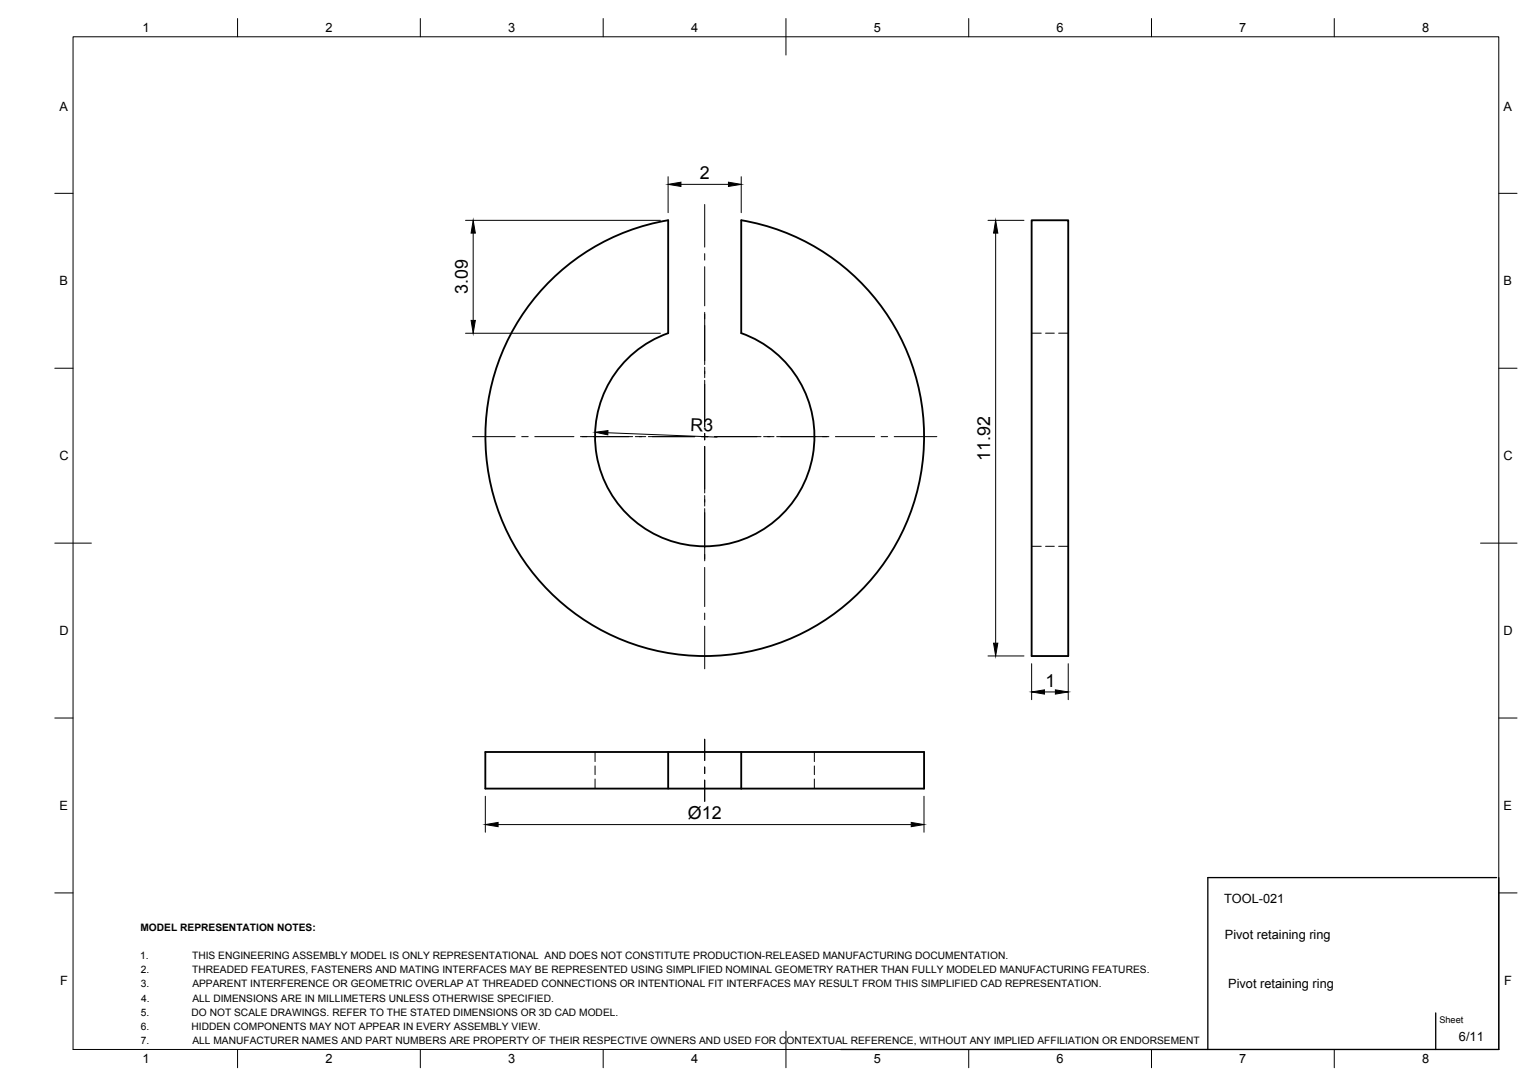
ISO-10303-21;
HEADER;
/* Generated by software containing ST-Developer
 * from STEP Tools, Inc. (www.steptools.com) 
 */

FILE_DESCRIPTION(
/* description */ (''),
/* implementation_level */ '2;1');

FILE_NAME(
/* name */ 'Pivot retaining ring.step',
/* time_stamp */ '2026-11-10T09:05:57-08:00',
/* author */ (''),
/* organization */ (''),
/* preprocessor_version */ 'ST-DEVELOPER v20.2',
/* originating_system */ 'Autodesk Translation Framework v15.17.0.0',
/* authorisation */ '');

FILE_SCHEMA (('AUTOMOTIVE_DESIGN { 1 0 10303 214 3 1 1 }'));
ENDSEC;

DATA;
#10=MECHANICAL_DESIGN_GEOMETRIC_PRESENTATION_REPRESENTATION('',(#568),#19618);
#548=SHAPE_REPRESENTATION_RELATIONSHIP('SRR','None',#19667,#558);
#558=ADVANCED_BREP_SHAPE_REPRESENTATION('',(#578),#19610);
#568=STYLED_ITEM('',(#19730),#578);
#578=MANIFOLD_SOLID_BREP('Body1',#7106);
#703=PLANE('',#7362);
#704=PLANE('',#7363);
#705=PLANE('',#7364);
#706=PLANE('',#7371);
#892=FACE_OUTER_BOUND('',#1314,.T.);
#893=FACE_OUTER_BOUND('',#1315,.T.);
#894=FACE_OUTER_BOUND('',#1316,.T.);
#895=FACE_OUTER_BOUND('',#1317,.T.);
#896=FACE_OUTER_BOUND('',#1318,.T.);
#897=FACE_OUTER_BOUND('',#1319,.T.);
#1314=EDGE_LOOP('',(#4866,#4867,#4868,#4869));
#1315=EDGE_LOOP('',(#4870,#4871,#4872,#4873));
#1316=EDGE_LOOP('',(#4874,#4875,#4876,#4877));
#1317=EDGE_LOOP('',(#4878,#4879,#4880,#4881));
#1318=EDGE_LOOP('',(#4882,#4883,#4884,#4885));
#1319=EDGE_LOOP('',(#4886,#4887,#4888,#4889));
#1817=LINE('',#9697,#2276);
#1818=LINE('',#9699,#2277);
#1819=LINE('',#9701,#2278);
#1820=LINE('',#9702,#2279);
#1821=LINE('',#9706,#2280);
#1822=LINE('',#9708,#2281);
#1823=LINE('',#9710,#2282);
#1824=LINE('',#9711,#2283);
#2276=VECTOR('',#8166,1.);
#2277=VECTOR('',#8167,1.);
#2278=VECTOR('',#8168,1.);
#2279=VECTOR('',#8169,1.);
#2280=VECTOR('',#8172,1.);
#2281=VECTOR('',#8173,1.);
#2282=VECTOR('',#8174,1.);
#2283=VECTOR('',#8175,1.);
#2678=CIRCLE('',#7365,0.6);
#2679=CIRCLE('',#7366,0.3);
#2680=CIRCLE('',#7368,0.3);
#2681=CIRCLE('',#7370,0.6);
#2929=VERTEX_POINT('',#9695);
#2930=VERTEX_POINT('',#9696);
#2931=VERTEX_POINT('',#9698);
#2932=VERTEX_POINT('',#9700);
#2933=VERTEX_POINT('',#9704);
#2934=VERTEX_POINT('',#9705);
#2935=VERTEX_POINT('',#9707);
#2936=VERTEX_POINT('',#9709);
#3658=EDGE_CURVE('',#2929,#2930,#1817,.T.);
#3659=EDGE_CURVE('',#2931,#2929,#1818,.T.);
#3660=EDGE_CURVE('',#2932,#2931,#1819,.T.);
#3661=EDGE_CURVE('',#2930,#2932,#1820,.T.);
#3662=EDGE_CURVE('',#2933,#2934,#1821,.T.);
#3663=EDGE_CURVE('',#2935,#2933,#1822,.T.);
#3664=EDGE_CURVE('',#2936,#2935,#1823,.T.);
#3665=EDGE_CURVE('',#2934,#2936,#1824,.T.);
#3666=EDGE_CURVE('',#2931,#2936,#2678,.T.);
#3667=EDGE_CURVE('',#2934,#2929,#2679,.T.);
#3668=EDGE_CURVE('',#2933,#2930,#2680,.T.);
#3669=EDGE_CURVE('',#2932,#2935,#2681,.T.);
#4866=ORIENTED_EDGE('',*,*,#3658,.F.);
#4867=ORIENTED_EDGE('',*,*,#3659,.F.);
#4868=ORIENTED_EDGE('',*,*,#3660,.F.);
#4869=ORIENTED_EDGE('',*,*,#3661,.F.);
#4870=ORIENTED_EDGE('',*,*,#3662,.F.);
#4871=ORIENTED_EDGE('',*,*,#3663,.F.);
#4872=ORIENTED_EDGE('',*,*,#3664,.F.);
#4873=ORIENTED_EDGE('',*,*,#3665,.F.);
#4874=ORIENTED_EDGE('',*,*,#3665,.T.);
#4875=ORIENTED_EDGE('',*,*,#3666,.F.);
#4876=ORIENTED_EDGE('',*,*,#3659,.T.);
#4877=ORIENTED_EDGE('',*,*,#3667,.F.);
#4878=ORIENTED_EDGE('',*,*,#3662,.T.);
#4879=ORIENTED_EDGE('',*,*,#3667,.T.);
#4880=ORIENTED_EDGE('',*,*,#3658,.T.);
#4881=ORIENTED_EDGE('',*,*,#3668,.F.);
#4882=ORIENTED_EDGE('',*,*,#3664,.T.);
#4883=ORIENTED_EDGE('',*,*,#3669,.F.);
#4884=ORIENTED_EDGE('',*,*,#3660,.T.);
#4885=ORIENTED_EDGE('',*,*,#3666,.T.);
#4886=ORIENTED_EDGE('',*,*,#3663,.T.);
#4887=ORIENTED_EDGE('',*,*,#3668,.T.);
#4888=ORIENTED_EDGE('',*,*,#3661,.T.);
#4889=ORIENTED_EDGE('',*,*,#3669,.T.);
#6583=CYLINDRICAL_SURFACE('',#7367,0.3);
#6584=CYLINDRICAL_SURFACE('',#7369,0.6);
#6771=ADVANCED_FACE('',(#892),#703,.F.);
#6772=ADVANCED_FACE('',(#893),#704,.F.);
#6773=ADVANCED_FACE('',(#894),#705,.F.);
#6774=ADVANCED_FACE('',(#895),#6583,.F.);
#6775=ADVANCED_FACE('',(#896),#6584,.T.);
#6776=ADVANCED_FACE('',(#897),#706,.T.);
#7106=CLOSED_SHELL('',(#6771,#6772,#6773,#6774,#6775,#6776));
#7361=AXIS2_PLACEMENT_3D('',#9693,#8162,#8163);
#7362=AXIS2_PLACEMENT_3D('',#9694,#8164,#8165);
#7363=AXIS2_PLACEMENT_3D('',#9703,#8170,#8171);
#7364=AXIS2_PLACEMENT_3D('',#9712,#8176,#8177);
#7365=AXIS2_PLACEMENT_3D('',#9713,#8178,#8179);
#7366=AXIS2_PLACEMENT_3D('',#9714,#8180,#8181);
#7367=AXIS2_PLACEMENT_3D('',#9715,#8182,#8183);
#7368=AXIS2_PLACEMENT_3D('',#9716,#8184,#8185);
#7369=AXIS2_PLACEMENT_3D('',#9717,#8186,#8187);
#7370=AXIS2_PLACEMENT_3D('',#9718,#8188,#8189);
#7371=AXIS2_PLACEMENT_3D('',#9719,#8190,#8191);
#8162=DIRECTION('axis',(0.,0.,1.));
#8163=DIRECTION('refdir',(1.,0.,0.));
#8164=DIRECTION('center_axis',(-1.,0.,0.));
#8165=DIRECTION('ref_axis',(0.,1.,0.));
#8166=DIRECTION('',(0.,0.,1.));
#8167=DIRECTION('',(0.,-1.,0.));
#8168=DIRECTION('',(0.,0.,-1.));
#8169=DIRECTION('',(0.,1.,0.));
#8170=DIRECTION('center_axis',(1.,0.,0.));
#8171=DIRECTION('ref_axis',(0.,-1.,0.));
#8172=DIRECTION('',(0.,0.,-1.));
#8173=DIRECTION('',(0.,-1.,0.));
#8174=DIRECTION('',(0.,0.,1.));
#8175=DIRECTION('',(0.,1.,0.));
#8176=DIRECTION('center_axis',(0.,0.,1.));
#8177=DIRECTION('ref_axis',(1.,0.,0.));
#8178=DIRECTION('center_axis',(0.,0.,1.));
#8179=DIRECTION('ref_axis',(1.,0.,0.));
#8180=DIRECTION('center_axis',(0.,0.,-1.));
#8181=DIRECTION('ref_axis',(1.,0.,0.));
#8182=DIRECTION('center_axis',(0.,0.,1.));
#8183=DIRECTION('ref_axis',(6.12323399573677E-17,-1.,0.));
#8184=DIRECTION('center_axis',(0.,0.,-1.));
#8185=DIRECTION('ref_axis',(1.,0.,0.));
#8186=DIRECTION('center_axis',(0.,0.,1.));
#8187=DIRECTION('ref_axis',(6.12323399573677E-17,-1.,0.));
#8188=DIRECTION('center_axis',(0.,0.,1.));
#8189=DIRECTION('ref_axis',(1.,0.,0.));
#8190=DIRECTION('center_axis',(0.,0.,1.));
#8191=DIRECTION('ref_axis',(1.,0.,0.));
#9693=CARTESIAN_POINT('',(0.,0.,0.));
#9694=CARTESIAN_POINT('Origin',(-0.1,0.,0.1));
#9695=CARTESIAN_POINT('',(-0.1,0.282842712474619,0.));
#9696=CARTESIAN_POINT('',(-0.1,0.282842712474619,0.1));
#9697=CARTESIAN_POINT('',(-0.1,0.282842712474619,0.));
#9698=CARTESIAN_POINT('',(-0.1,0.591607978309962,0.));
#9699=CARTESIAN_POINT('',(-0.1,0.,0.));
#9700=CARTESIAN_POINT('',(-0.1,0.591607978309962,0.1));
#9701=CARTESIAN_POINT('',(-0.1,0.591607978309962,0.));
#9702=CARTESIAN_POINT('',(-0.1,0.,0.1));
#9703=CARTESIAN_POINT('Origin',(0.1,1.2,0.1));
#9704=CARTESIAN_POINT('',(0.1,0.282842712474619,0.1));
#9705=CARTESIAN_POINT('',(0.1,0.282842712474619,0.));
#9706=CARTESIAN_POINT('',(0.1,0.282842712474619,0.));
#9707=CARTESIAN_POINT('',(0.1,0.591607978309962,0.1));
#9708=CARTESIAN_POINT('',(0.1,0.6,0.1));
#9709=CARTESIAN_POINT('',(0.1,0.591607978309962,0.));
#9710=CARTESIAN_POINT('',(0.1,0.591607978309962,0.));
#9711=CARTESIAN_POINT('',(0.1,0.6,0.));
#9712=CARTESIAN_POINT('Origin',(0.,0.,0.));
#9713=CARTESIAN_POINT('Origin',(0.,0.,0.));
#9714=CARTESIAN_POINT('Origin',(0.,0.,0.));
#9715=CARTESIAN_POINT('Origin',(0.,0.,0.));
#9716=CARTESIAN_POINT('Origin',(0.,0.,0.1));
#9717=CARTESIAN_POINT('Origin',(0.,0.,0.));
#9718=CARTESIAN_POINT('Origin',(0.,0.,0.1));
#9719=CARTESIAN_POINT('Origin',(0.,0.,0.1));
#19597=UNCERTAINTY_MEASURE_WITH_UNIT(LENGTH_MEASURE(0.001),#19619,
'DISTANCE_ACCURACY_VALUE',
'Maximum model space distance between geometric entities at asserted c
onnectivities');
#19605=UNCERTAINTY_MEASURE_WITH_UNIT(LENGTH_MEASURE(0.001),#19619,
'DISTANCE_ACCURACY_VALUE',
'Maximum model space distance between geometric entities at asserted c
onnectivities');
#19610=(
GEOMETRIC_REPRESENTATION_CONTEXT(3)
GLOBAL_UNCERTAINTY_ASSIGNED_CONTEXT((#19597))
GLOBAL_UNIT_ASSIGNED_CONTEXT((#19619,#19621,#19622))
REPRESENTATION_CONTEXT('','3D')
);
#19618=(
GEOMETRIC_REPRESENTATION_CONTEXT(3)
GLOBAL_UNCERTAINTY_ASSIGNED_CONTEXT((#19605))
GLOBAL_UNIT_ASSIGNED_CONTEXT((#19619,#19621,#19622))
REPRESENTATION_CONTEXT('','3D')
);
#19619=(
LENGTH_UNIT()
NAMED_UNIT(*)
SI_UNIT(.CENTI.,.METRE.)
);
#19621=(
NAMED_UNIT(*)
PLANE_ANGLE_UNIT()
SI_UNIT($,.RADIAN.)
);
#19622=(
NAMED_UNIT(*)
SI_UNIT($,.STERADIAN.)
SOLID_ANGLE_UNIT()
);
#19627=SHAPE_DEFINITION_REPRESENTATION(#19639,#19667);
#19639=PRODUCT_DEFINITION_SHAPE('',$,#19680);
#19667=SHAPE_REPRESENTATION('',(#7361),#19610);
#19675=PRODUCT_DEFINITION_CONTEXT('part definition',#19713,'design');
#19680=PRODUCT_DEFINITION('Pivot retaining ring','Pivot retaining ring',
#19692,#19675);
#19692=PRODUCT_DEFINITION_FORMATION('',$,#19719);
#19713=APPLICATION_CONTEXT(
'Core Data for Automotive Mechanical Design Process');
#19714=PRODUCT_CONTEXT('part definition',#19713,'mechanical');
#19719=PRODUCT('Pivot retaining ring','Pivot retaining ring',$,(#19714));
#19730=PRESENTATION_STYLE_ASSIGNMENT((#19738));
#19738=SURFACE_STYLE_USAGE(.BOTH.,#19746);
#19746=SURFACE_SIDE_STYLE('',(#19754));
#19754=SURFACE_STYLE_FILL_AREA(#19762);
#19762=FILL_AREA_STYLE('Dark gray',(#19770));
#19770=FILL_AREA_STYLE_COLOUR('Dark gray',#19778);
#19778=COLOUR_RGB('Dark gray',0.250980392156863,0.282352941176471,0.32156862745098);
ENDSEC;
END-ISO-10303-21;
